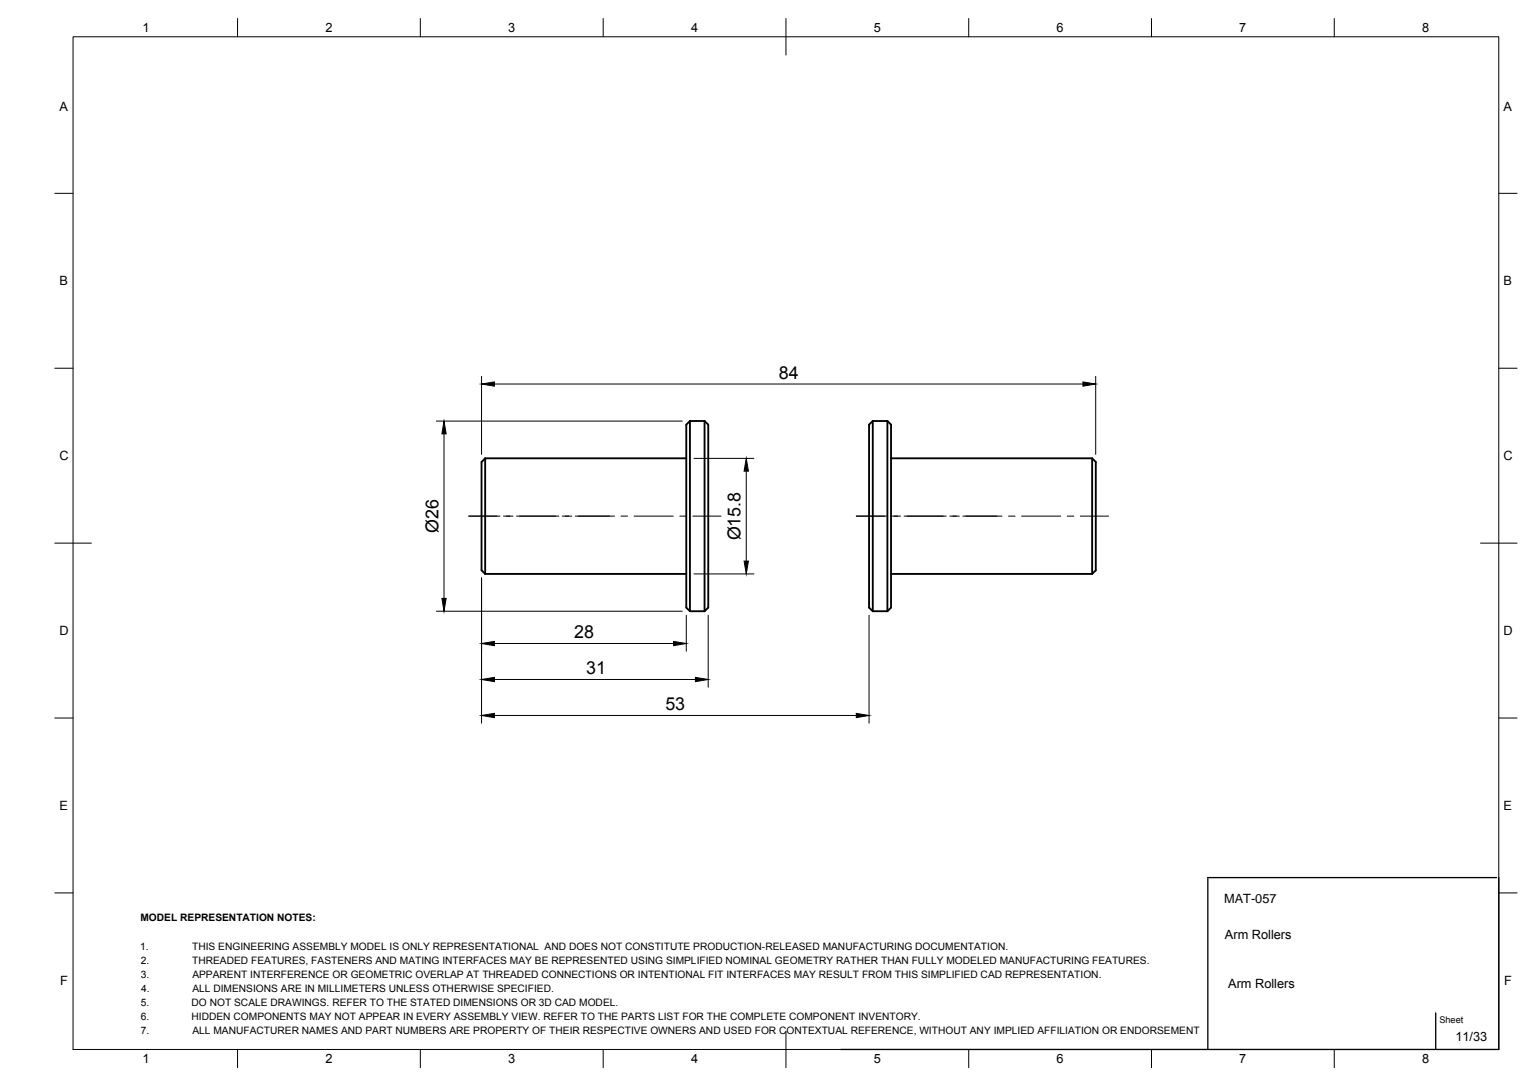
ISO-10303-21;
HEADER;
/* Generated by software containing ST-Developer
 * from STEP Tools, Inc. (www.steptools.com) 
 */

FILE_DESCRIPTION(
/* description */ ('STEP AP214', 'CAx-IF Rec.Pracs.---Representation and Presentation of Product Manufa
cturing Information (PMI)---4.0---2014-10-13'),
/* implementation_level */ '2;1');

FILE_NAME(
/* name */ 'Arm Rollers.step',
/* time_stamp */ '2026-10-28T23:34:22+01:00',
/* author */ (''),
/* organization */ (''),
/* preprocessor_version */ 'ST-DEVELOPER v20.2',
/* originating_system */ 'Autodesk Translation Framework v15.17.0.0',
/* authorisation */ '');

FILE_SCHEMA (('AP242_MANAGED_MODEL_BASED_3D_ENGINEERING_MIM_LF { 1 0 10303 442 2 1 4 }'));
ENDSEC;

DATA;
#10=MECHANICAL_DESIGN_GEOMETRIC_PRESENTATION_REPRESENTATION('',(#252,#253),#27807);
#208=SHAPE_REPRESENTATION_RELATIONSHIP('SRR','None',#27903,#230);
#230=ADVANCED_BREP_SHAPE_REPRESENTATION('',(#281,#282),#27783);
#252=STYLED_ITEM('',(#28063),#281);
#253=STYLED_ITEM('',(#28063),#282);
#281=MANIFOLD_SOLID_BREP('Body1',#12028);
#282=MANIFOLD_SOLID_BREP('Body2',#12029);
#375=FACE_BOUND('',#2200,.T.);
#376=FACE_BOUND('',#2209,.T.);
#536=PLANE('',#12763);
#537=PLANE('',#12764);
#538=PLANE('',#12765);
#539=PLANE('',#12779);
#540=PLANE('',#12780);
#541=PLANE('',#12781);
#1068=CYLINDRICAL_SURFACE('',#12760,7.89999999999999);
#1069=CYLINDRICAL_SURFACE('',#12762,13.);
#1070=CYLINDRICAL_SURFACE('',#12776,7.89999999999999);
#1071=CYLINDRICAL_SURFACE('',#12778,13.);
#1456=FACE_OUTER_BOUND('',#2193,.T.);
#1457=FACE_OUTER_BOUND('',#2194,.T.);
#1458=FACE_OUTER_BOUND('',#2195,.T.);
#1459=FACE_OUTER_BOUND('',#2196,.T.);
#1460=FACE_OUTER_BOUND('',#2197,.T.);
#1461=FACE_OUTER_BOUND('',#2198,.T.);
#1462=FACE_OUTER_BOUND('',#2199,.T.);
#1463=FACE_OUTER_BOUND('',#2201,.T.);
#1464=FACE_OUTER_BOUND('',#2202,.T.);
#1465=FACE_OUTER_BOUND('',#2203,.T.);
#1466=FACE_OUTER_BOUND('',#2204,.T.);
#1467=FACE_OUTER_BOUND('',#2205,.T.);
#1468=FACE_OUTER_BOUND('',#2206,.T.);
#1469=FACE_OUTER_BOUND('',#2207,.T.);
#1470=FACE_OUTER_BOUND('',#2208,.T.);
#1471=FACE_OUTER_BOUND('',#2210,.T.);
#2193=EDGE_LOOP('',(#8961,#8962,#8963,#8964));
#2194=EDGE_LOOP('',(#8965,#8966,#8967,#8968));
#2195=EDGE_LOOP('',(#8969,#8970,#8971,#8972,#8973));
#2196=EDGE_LOOP('',(#8974,#8975,#8976,#8977));
#2197=EDGE_LOOP('',(#8978,#8979,#8980,#8981,#8982));
#2198=EDGE_LOOP('',(#8983));
#2199=EDGE_LOOP('',(#8984));
#2200=EDGE_LOOP('',(#8985));
#2201=EDGE_LOOP('',(#8986));
#2202=EDGE_LOOP('',(#8987,#8988,#8989,#8990));
#2203=EDGE_LOOP('',(#8991,#8992,#8993,#8994));
#2204=EDGE_LOOP('',(#8995,#8996,#8997,#8998,#8999));
#2205=EDGE_LOOP('',(#9000,#9001,#9002,#9003));
#2206=EDGE_LOOP('',(#9004,#9005,#9006,#9007,#9008));
#2207=EDGE_LOOP('',(#9009));
#2208=EDGE_LOOP('',(#9010));
#2209=EDGE_LOOP('',(#9011));
#2210=EDGE_LOOP('',(#9012));
#3045=LINE('',#18795,#3865);
#3046=LINE('',#18801,#3866);
#3047=LINE('',#18809,#3867);
#3048=LINE('',#18814,#3868);
#3049=LINE('',#18816,#3869);
#3050=LINE('',#18824,#3870);
#3051=LINE('',#18830,#3871);
#3052=LINE('',#18837,#3872);
#3053=LINE('',#18843,#3873);
#3054=LINE('',#18845,#3874);
#3865=VECTOR('',#14931,7.39999999999998);
#3866=VECTOR('',#14938,12.5);
#3867=VECTOR('',#14947,13.);
#3868=VECTOR('',#14954,7.89999999999999);
#3869=VECTOR('',#14957,13.);
#3870=VECTOR('',#14968,7.39999999999998);
#3871=VECTOR('',#14975,12.5);
#3872=VECTOR('',#14982,13.);
#3873=VECTOR('',#14991,7.89999999999999);
#3874=VECTOR('',#14994,13.);
#4609=CIRCLE('',#12751,7.89999999999999);
#4610=CIRCLE('',#12752,7.39999999999998);
#4611=CIRCLE('',#12754,13.);
#4612=CIRCLE('',#12755,12.5);
#4613=CIRCLE('',#12757,13.);
#4614=CIRCLE('',#12758,13.);
#4615=CIRCLE('',#12759,12.5);
#4616=CIRCLE('',#12761,7.89999999999999);
#4617=CIRCLE('',#12767,7.89999999999999);
#4618=CIRCLE('',#12768,7.39999999999998);
#4619=CIRCLE('',#12770,13.);
#4620=CIRCLE('',#12771,12.5);
#4621=CIRCLE('',#12773,13.);
#4622=CIRCLE('',#12774,12.5);
#4623=CIRCLE('',#12775,13.);
#4624=CIRCLE('',#12777,7.89999999999999);
#5393=VERTEX_POINT('',#18792);
#5394=VERTEX_POINT('',#18794);
#5395=VERTEX_POINT('',#18798);
#5396=VERTEX_POINT('',#18800);
#5397=VERTEX_POINT('',#18804);
#5398=VERTEX_POINT('',#18805);
#5399=VERTEX_POINT('',#18808);
#5400=VERTEX_POINT('',#18812);
#5401=VERTEX_POINT('',#18821);
#5402=VERTEX_POINT('',#18823);
#5403=VERTEX_POINT('',#18827);
#5404=VERTEX_POINT('',#18829);
#5405=VERTEX_POINT('',#18833);
#5406=VERTEX_POINT('',#18834);
#5407=VERTEX_POINT('',#18836);
#5408=VERTEX_POINT('',#18841);
#6693=EDGE_CURVE('',#5393,#5393,#4609,.T.);
#6694=EDGE_CURVE('',#5393,#5394,#3045,.T.);
#6695=EDGE_CURVE('',#5394,#5394,#4610,.T.);
#6696=EDGE_CURVE('',#5395,#5395,#4611,.T.);
#6697=EDGE_CURVE('',#5395,#5396,#3046,.T.);
#6698=EDGE_CURVE('',#5396,#5396,#4612,.T.);
#6699=EDGE_CURVE('',#5397,#5398,#4613,.T.);
#6700=EDGE_CURVE('',#5398,#5397,#4614,.T.);
#6701=EDGE_CURVE('',#5398,#5399,#3047,.T.);
#6702=EDGE_CURVE('',#5399,#5399,#4615,.T.);
#6703=EDGE_CURVE('',#5400,#5400,#4616,.T.);
#6704=EDGE_CURVE('',#5400,#5393,#3048,.T.);
#6705=EDGE_CURVE('',#5397,#5395,#3049,.T.);
#6706=EDGE_CURVE('',#5401,#5401,#4617,.T.);
#6707=EDGE_CURVE('',#5401,#5402,#3050,.T.);
#6708=EDGE_CURVE('',#5402,#5402,#4618,.T.);
#6709=EDGE_CURVE('',#5403,#5403,#4619,.T.);
#6710=EDGE_CURVE('',#5403,#5404,#3051,.T.);
#6711=EDGE_CURVE('',#5404,#5404,#4620,.T.);
#6712=EDGE_CURVE('',#5405,#5406,#4621,.T.);
#6713=EDGE_CURVE('',#5406,#5407,#3052,.T.);
#6714=EDGE_CURVE('',#5407,#5407,#4622,.T.);
#6715=EDGE_CURVE('',#5406,#5405,#4623,.T.);
#6716=EDGE_CURVE('',#5408,#5408,#4624,.T.);
#6717=EDGE_CURVE('',#5408,#5401,#3053,.T.);
#6718=EDGE_CURVE('',#5405,#5403,#3054,.T.);
#8961=ORIENTED_EDGE('',*,*,#6693,.F.);
#8962=ORIENTED_EDGE('',*,*,#6694,.T.);
#8963=ORIENTED_EDGE('',*,*,#6695,.F.);
#8964=ORIENTED_EDGE('',*,*,#6694,.F.);
#8965=ORIENTED_EDGE('',*,*,#6696,.F.);
#8966=ORIENTED_EDGE('',*,*,#6697,.T.);
#8967=ORIENTED_EDGE('',*,*,#6698,.F.);
#8968=ORIENTED_EDGE('',*,*,#6697,.F.);
#8969=ORIENTED_EDGE('',*,*,#6699,.F.);
#8970=ORIENTED_EDGE('',*,*,#6700,.F.);
#8971=ORIENTED_EDGE('',*,*,#6701,.T.);
#8972=ORIENTED_EDGE('',*,*,#6702,.F.);
#8973=ORIENTED_EDGE('',*,*,#6701,.F.);
#8974=ORIENTED_EDGE('',*,*,#6703,.T.);
#8975=ORIENTED_EDGE('',*,*,#6704,.T.);
#8976=ORIENTED_EDGE('',*,*,#6693,.T.);
#8977=ORIENTED_EDGE('',*,*,#6704,.F.);
#8978=ORIENTED_EDGE('',*,*,#6699,.T.);
#8979=ORIENTED_EDGE('',*,*,#6700,.T.);
#8980=ORIENTED_EDGE('',*,*,#6705,.T.);
#8981=ORIENTED_EDGE('',*,*,#6696,.T.);
#8982=ORIENTED_EDGE('',*,*,#6705,.F.);
#8983=ORIENTED_EDGE('',*,*,#6698,.T.);
#8984=ORIENTED_EDGE('',*,*,#6702,.T.);
#8985=ORIENTED_EDGE('',*,*,#6703,.F.);
#8986=ORIENTED_EDGE('',*,*,#6695,.T.);
#8987=ORIENTED_EDGE('',*,*,#6706,.T.);
#8988=ORIENTED_EDGE('',*,*,#6707,.T.);
#8989=ORIENTED_EDGE('',*,*,#6708,.T.);
#8990=ORIENTED_EDGE('',*,*,#6707,.F.);
#8991=ORIENTED_EDGE('',*,*,#6709,.T.);
#8992=ORIENTED_EDGE('',*,*,#6710,.T.);
#8993=ORIENTED_EDGE('',*,*,#6711,.T.);
#8994=ORIENTED_EDGE('',*,*,#6710,.F.);
#8995=ORIENTED_EDGE('',*,*,#6712,.T.);
#8996=ORIENTED_EDGE('',*,*,#6713,.T.);
#8997=ORIENTED_EDGE('',*,*,#6714,.T.);
#8998=ORIENTED_EDGE('',*,*,#6713,.F.);
#8999=ORIENTED_EDGE('',*,*,#6715,.T.);
#9000=ORIENTED_EDGE('',*,*,#6716,.F.);
#9001=ORIENTED_EDGE('',*,*,#6717,.T.);
#9002=ORIENTED_EDGE('',*,*,#6706,.F.);
#9003=ORIENTED_EDGE('',*,*,#6717,.F.);
#9004=ORIENTED_EDGE('',*,*,#6712,.F.);
#9005=ORIENTED_EDGE('',*,*,#6718,.T.);
#9006=ORIENTED_EDGE('',*,*,#6709,.F.);
#9007=ORIENTED_EDGE('',*,*,#6718,.F.);
#9008=ORIENTED_EDGE('',*,*,#6715,.F.);
#9009=ORIENTED_EDGE('',*,*,#6711,.F.);
#9010=ORIENTED_EDGE('',*,*,#6714,.F.);
#9011=ORIENTED_EDGE('',*,*,#6716,.T.);
#9012=ORIENTED_EDGE('',*,*,#6708,.F.);
#11285=CONICAL_SURFACE('',#12750,7.39999999999998,0.785398163397459);
#11286=CONICAL_SURFACE('',#12753,12.5,0.785398163397438);
#11287=CONICAL_SURFACE('',#12756,13.,0.785398163397455);
#11288=CONICAL_SURFACE('',#12766,7.39999999999998,0.785398163397459);
#11289=CONICAL_SURFACE('',#12769,12.5,0.785398163397438);
#11290=CONICAL_SURFACE('',#12772,13.,0.785398163397455);
#11538=ADVANCED_FACE('',(#1456),#11285,.T.);
#11539=ADVANCED_FACE('',(#1457),#11286,.T.);
#11540=ADVANCED_FACE('',(#1458),#11287,.T.);
#11541=ADVANCED_FACE('',(#1459),#1068,.T.);
#11542=ADVANCED_FACE('',(#1460),#1069,.T.);
#11543=ADVANCED_FACE('',(#1461),#536,.T.);
#11544=ADVANCED_FACE('',(#1462,#375),#537,.F.);
#11545=ADVANCED_FACE('',(#1463),#538,.T.);
#11546=ADVANCED_FACE('',(#1464),#11288,.T.);
#11547=ADVANCED_FACE('',(#1465),#11289,.T.);
#11548=ADVANCED_FACE('',(#1466),#11290,.T.);
#11549=ADVANCED_FACE('',(#1467),#1070,.T.);
#11550=ADVANCED_FACE('',(#1468),#1071,.T.);
#11551=ADVANCED_FACE('',(#1469),#539,.T.);
#11552=ADVANCED_FACE('',(#1470,#376),#540,.F.);
#11553=ADVANCED_FACE('',(#1471),#541,.T.);
#12028=CLOSED_SHELL('',(#11538,#11539,#11540,#11541,#11542,#11543,#11544,
#11545));
#12029=CLOSED_SHELL('',(#11546,#11547,#11548,#11549,#11550,#11551,#11552,
#11553));
#12749=AXIS2_PLACEMENT_3D('',#18790,#14925,#14926);
#12750=AXIS2_PLACEMENT_3D('',#18791,#14927,#14928);
#12751=AXIS2_PLACEMENT_3D('',#18793,#14929,#14930);
#12752=AXIS2_PLACEMENT_3D('',#18796,#14932,#14933);
#12753=AXIS2_PLACEMENT_3D('',#18797,#14934,#14935);
#12754=AXIS2_PLACEMENT_3D('',#18799,#14936,#14937);
#12755=AXIS2_PLACEMENT_3D('',#18802,#14939,#14940);
#12756=AXIS2_PLACEMENT_3D('',#18803,#14941,#14942);
#12757=AXIS2_PLACEMENT_3D('',#18806,#14943,#14944);
#12758=AXIS2_PLACEMENT_3D('',#18807,#14945,#14946);
#12759=AXIS2_PLACEMENT_3D('',#18810,#14948,#14949);
#12760=AXIS2_PLACEMENT_3D('',#18811,#14950,#14951);
#12761=AXIS2_PLACEMENT_3D('',#18813,#14952,#14953);
#12762=AXIS2_PLACEMENT_3D('',#18815,#14955,#14956);
#12763=AXIS2_PLACEMENT_3D('',#18817,#14958,#14959);
#12764=AXIS2_PLACEMENT_3D('',#18818,#14960,#14961);
#12765=AXIS2_PLACEMENT_3D('',#18819,#14962,#14963);
#12766=AXIS2_PLACEMENT_3D('',#18820,#14964,#14965);
#12767=AXIS2_PLACEMENT_3D('',#18822,#14966,#14967);
#12768=AXIS2_PLACEMENT_3D('',#18825,#14969,#14970);
#12769=AXIS2_PLACEMENT_3D('',#18826,#14971,#14972);
#12770=AXIS2_PLACEMENT_3D('',#18828,#14973,#14974);
#12771=AXIS2_PLACEMENT_3D('',#18831,#14976,#14977);
#12772=AXIS2_PLACEMENT_3D('',#18832,#14978,#14979);
#12773=AXIS2_PLACEMENT_3D('',#18835,#14980,#14981);
#12774=AXIS2_PLACEMENT_3D('',#18838,#14983,#14984);
#12775=AXIS2_PLACEMENT_3D('',#18839,#14985,#14986);
#12776=AXIS2_PLACEMENT_3D('',#18840,#14987,#14988);
#12777=AXIS2_PLACEMENT_3D('',#18842,#14989,#14990);
#12778=AXIS2_PLACEMENT_3D('',#18844,#14992,#14993);
#12779=AXIS2_PLACEMENT_3D('',#18846,#14995,#14996);
#12780=AXIS2_PLACEMENT_3D('',#18847,#14997,#14998);
#12781=AXIS2_PLACEMENT_3D('',#18848,#14999,#15000);
#14925=DIRECTION('axis',(0.,0.,1.));
#14926=DIRECTION('refdir',(1.,0.,0.));
#14927=DIRECTION('center_axis',(0.,0.,1.));
#14928=DIRECTION('ref_axis',(1.,0.,0.));
#14929=DIRECTION('center_axis',(0.,0.,1.));
#14930=DIRECTION('ref_axis',(-1.,0.,0.));
#14931=DIRECTION('',(0.707106781186555,8.65956056235502E-17,-0.70710678118654));
#14932=DIRECTION('center_axis',(0.,0.,-1.));
#14933=DIRECTION('ref_axis',(-1.,0.,0.));
#14934=DIRECTION('center_axis',(0.,0.,-1.));
#14935=DIRECTION('ref_axis',(-1.,0.,0.));
#14936=DIRECTION('center_axis',(0.,0.,-1.));
#14937=DIRECTION('ref_axis',(1.,0.,0.));
#14938=DIRECTION('',(-0.70710678118654,8.65956056235484E-17,0.707106781186555));
#14939=DIRECTION('center_axis',(0.,0.,1.));
#14940=DIRECTION('ref_axis',(1.,0.,0.));
#14941=DIRECTION('center_axis',(0.,0.,1.));
#14942=DIRECTION('ref_axis',(1.,0.,0.));
#14943=DIRECTION('center_axis',(0.,0.,1.));
#14944=DIRECTION('ref_axis',(1.,0.,0.));
#14945=DIRECTION('center_axis',(0.,0.,1.));
#14946=DIRECTION('ref_axis',(1.,0.,0.));
#14947=DIRECTION('',(0.707106781186552,8.65956056235499E-17,-0.707106781186543));
#14948=DIRECTION('center_axis',(0.,0.,-1.));
#14949=DIRECTION('ref_axis',(1.,0.,0.));
#14950=DIRECTION('center_axis',(0.,0.,1.));
#14951=DIRECTION('ref_axis',(1.,0.,0.));
#14952=DIRECTION('center_axis',(0.,0.,-1.));
#14953=DIRECTION('ref_axis',(-1.,0.,0.));
#14954=DIRECTION('',(0.,0.,-1.));
#14955=DIRECTION('center_axis',(0.,0.,-1.));
#14956=DIRECTION('ref_axis',(-1.,0.,0.));
#14957=DIRECTION('',(0.,0.,1.));
#14958=DIRECTION('center_axis',(0.,0.,1.));
#14959=DIRECTION('ref_axis',(1.,0.,0.));
#14960=DIRECTION('center_axis',(0.,0.,1.));
#14961=DIRECTION('ref_axis',(1.,0.,0.));
#14962=DIRECTION('center_axis',(0.,0.,-1.));
#14963=DIRECTION('ref_axis',(1.,0.,0.));
#14964=DIRECTION('center_axis',(0.,0.,-1.));
#14965=DIRECTION('ref_axis',(1.,0.,0.));
#14966=DIRECTION('center_axis',(0.,0.,1.));
#14967=DIRECTION('ref_axis',(-1.,0.,0.));
#14968=DIRECTION('',(0.707106781186555,-8.65956056235502E-17,0.70710678118654));
#14969=DIRECTION('center_axis',(0.,0.,-1.));
#14970=DIRECTION('ref_axis',(-1.,0.,0.));
#14971=DIRECTION('center_axis',(0.,0.,1.));
#14972=DIRECTION('ref_axis',(-1.,0.,0.));
#14973=DIRECTION('center_axis',(0.,0.,-1.));
#14974=DIRECTION('ref_axis',(1.,0.,0.));
#14975=DIRECTION('',(-0.70710678118654,-8.65956056235484E-17,-0.707106781186555));
#14976=DIRECTION('center_axis',(0.,0.,1.));
#14977=DIRECTION('ref_axis',(1.,0.,0.));
#14978=DIRECTION('center_axis',(0.,0.,-1.));
#14979=DIRECTION('ref_axis',(1.,0.,0.));
#14980=DIRECTION('center_axis',(0.,0.,1.));
#14981=DIRECTION('ref_axis',(1.,0.,0.));
#14982=DIRECTION('',(0.707106781186552,-8.65956056235499E-17,0.707106781186543));
#14983=DIRECTION('center_axis',(0.,0.,-1.));
#14984=DIRECTION('ref_axis',(1.,0.,0.));
#14985=DIRECTION('center_axis',(0.,0.,1.));
#14986=DIRECTION('ref_axis',(1.,0.,0.));
#14987=DIRECTION('center_axis',(0.,0.,-1.));
#14988=DIRECTION('ref_axis',(1.,0.,0.));
#14989=DIRECTION('center_axis',(0.,0.,-1.));
#14990=DIRECTION('ref_axis',(-1.,0.,0.));
#14991=DIRECTION('',(0.,0.,1.));
#14992=DIRECTION('center_axis',(0.,0.,1.));
#14993=DIRECTION('ref_axis',(-1.,0.,0.));
#14994=DIRECTION('',(0.,0.,-1.));
#14995=DIRECTION('center_axis',(0.,0.,-1.));
#14996=DIRECTION('ref_axis',(1.,0.,0.));
#14997=DIRECTION('center_axis',(0.,0.,-1.));
#14998=DIRECTION('ref_axis',(1.,0.,0.));
#14999=DIRECTION('center_axis',(0.,0.,1.));
#15000=DIRECTION('ref_axis',(1.,0.,0.));
#18790=CARTESIAN_POINT('',(0.,0.,0.));
#18791=CARTESIAN_POINT('Origin',(37.0412526478464,187.739737607039,211.073593133701));
#18792=CARTESIAN_POINT('',(29.1412526478464,187.739737607039,211.573593133701));
#18793=CARTESIAN_POINT('Origin',(37.0412526478464,187.739737607039,211.573593133701));
#18794=CARTESIAN_POINT('',(29.6412526478464,187.739737607039,211.073593133701));
#18795=CARTESIAN_POINT('',(29.6412526478464,187.739737607039,211.073593133701));
#18796=CARTESIAN_POINT('Origin',(37.0412526478464,187.739737607039,211.073593133701));
#18797=CARTESIAN_POINT('Origin',(37.0412526479213,187.739737607024,242.073593133701));
#18798=CARTESIAN_POINT('',(50.0412526479213,187.739737607024,241.573593133701));
#18799=CARTESIAN_POINT('Origin',(37.0412526479213,187.739737607024,241.573593133701));
#18800=CARTESIAN_POINT('',(49.5412526479213,187.739737607024,242.073593133701));
#18801=CARTESIAN_POINT('',(49.5412526479213,187.739737607024,242.073593133701));
#18802=CARTESIAN_POINT('Origin',(37.0412526479213,187.739737607024,242.073593133701));
#18803=CARTESIAN_POINT('Origin',(37.0412526479213,187.739737607024,239.573593133701));
#18804=CARTESIAN_POINT('',(50.0412526479213,187.739737607024,239.573593133701));
#18805=CARTESIAN_POINT('',(24.0412526479213,187.739737607024,239.573593133701));
#18806=CARTESIAN_POINT('Origin',(37.0412526479213,187.739737607024,239.573593133701));
#18807=CARTESIAN_POINT('Origin',(37.0412526479213,187.739737607024,239.573593133701));
#18808=CARTESIAN_POINT('',(24.5412526479213,187.739737607024,239.073593133701));
#18809=CARTESIAN_POINT('',(24.0412526479213,187.739737607024,239.573593133701));
#18810=CARTESIAN_POINT('Origin',(37.0412526479213,187.739737607024,239.073593133701));
#18811=CARTESIAN_POINT('Origin',(37.0412526478464,187.739737607039,188.729018848206));
#18812=CARTESIAN_POINT('',(29.1412526478464,187.739737607039,239.073593133701));
#18813=CARTESIAN_POINT('Origin',(37.0412526478464,187.739737607039,239.073593133701));
#18814=CARTESIAN_POINT('',(29.1412526478464,187.739737607039,188.729018848206));
#18815=CARTESIAN_POINT('Origin',(37.0412526479213,187.739737607024,242.073593133701));
#18816=CARTESIAN_POINT('',(50.0412526479213,187.739737607024,242.073593133701));
#18817=CARTESIAN_POINT('Origin',(37.0412526479213,187.739737607024,242.073593133701));
#18818=CARTESIAN_POINT('Origin',(37.0412526479213,187.739737607024,239.073593133701));
#18819=CARTESIAN_POINT('Origin',(-276.958747352154,52.7397376070391,211.073593133701));
#18820=CARTESIAN_POINT('Origin',(37.0412526478464,187.739737607039,295.073593133701));
#18821=CARTESIAN_POINT('',(29.1412526478464,187.739737607039,294.573593133701));
#18822=CARTESIAN_POINT('Origin',(37.0412526478464,187.739737607039,294.573593133701));
#18823=CARTESIAN_POINT('',(29.6412526478464,187.739737607039,295.073593133701));
#18824=CARTESIAN_POINT('',(29.6412526478464,187.739737607039,295.073593133701));
#18825=CARTESIAN_POINT('Origin',(37.0412526478464,187.739737607039,295.073593133701));
#18826=CARTESIAN_POINT('Origin',(37.0412526479213,187.739737607024,264.073593133701));
#18827=CARTESIAN_POINT('',(50.0412526479213,187.739737607024,264.573593133701));
#18828=CARTESIAN_POINT('Origin',(37.0412526479213,187.739737607024,264.573593133701));
#18829=CARTESIAN_POINT('',(49.5412526479213,187.739737607024,264.073593133701));
#18830=CARTESIAN_POINT('',(49.5412526479213,187.739737607024,264.073593133701));
#18831=CARTESIAN_POINT('Origin',(37.0412526479213,187.739737607024,264.073593133701));
#18832=CARTESIAN_POINT('Origin',(37.0412526479213,187.739737607024,266.573593133701));
#18833=CARTESIAN_POINT('',(50.0412526479213,187.739737607024,266.573593133701));
#18834=CARTESIAN_POINT('',(24.0412526479213,187.739737607024,266.573593133701));
#18835=CARTESIAN_POINT('Origin',(37.0412526479213,187.739737607024,266.573593133701));
#18836=CARTESIAN_POINT('',(24.5412526479213,187.739737607024,267.073593133701));
#18837=CARTESIAN_POINT('',(24.0412526479213,187.739737607024,266.573593133701));
#18838=CARTESIAN_POINT('Origin',(37.0412526479213,187.739737607024,267.073593133701));
#18839=CARTESIAN_POINT('Origin',(37.0412526479213,187.739737607024,266.573593133701));
#18840=CARTESIAN_POINT('Origin',(37.0412526478464,187.739737607039,317.418167419196));
#18841=CARTESIAN_POINT('',(29.1412526478464,187.739737607039,267.073593133701));
#18842=CARTESIAN_POINT('Origin',(37.0412526478464,187.739737607039,267.073593133701));
#18843=CARTESIAN_POINT('',(29.1412526478464,187.739737607039,317.418167419196));
#18844=CARTESIAN_POINT('Origin',(37.0412526479213,187.739737607024,264.073593133701));
#18845=CARTESIAN_POINT('',(50.0412526479213,187.739737607024,264.073593133701));
#18846=CARTESIAN_POINT('Origin',(37.0412526479213,187.739737607024,264.073593133701));
#18847=CARTESIAN_POINT('Origin',(37.0412526479213,187.739737607024,267.073593133701));
#18848=CARTESIAN_POINT('Origin',(-276.958747352154,52.7397376070391,295.073593133701));
#27754=UNCERTAINTY_MEASURE_WITH_UNIT(LENGTH_MEASURE(0.01),#27808,
'DISTANCE_ACCURACY_VALUE',
'Maximum model space distance between geometric entities at asserted c
onnectivities');
#27778=UNCERTAINTY_MEASURE_WITH_UNIT(LENGTH_MEASURE(0.01),#27808,
'DISTANCE_ACCURACY_VALUE',
'Maximum model space distance between geometric entities at asserted c
onnectivities');
#27783=(
GEOMETRIC_REPRESENTATION_CONTEXT(3)
GLOBAL_UNCERTAINTY_ASSIGNED_CONTEXT((#27754))
GLOBAL_UNIT_ASSIGNED_CONTEXT((#27808,#27810,#27811))
REPRESENTATION_CONTEXT('','3D')
);
#27807=(
GEOMETRIC_REPRESENTATION_CONTEXT(3)
GLOBAL_UNCERTAINTY_ASSIGNED_CONTEXT((#27778))
GLOBAL_UNIT_ASSIGNED_CONTEXT((#27808,#27810,#27811))
REPRESENTATION_CONTEXT('','3D')
);
#27808=(
LENGTH_UNIT()
NAMED_UNIT(*)
SI_UNIT(.MILLI.,.METRE.)
);
#27810=(
NAMED_UNIT(*)
PLANE_ANGLE_UNIT()
SI_UNIT($,.RADIAN.)
);
#27811=(
NAMED_UNIT(*)
SI_UNIT($,.STERADIAN.)
SOLID_ANGLE_UNIT()
);
#27816=SHAPE_DEFINITION_REPRESENTATION(#27844,#27903);
#27844=PRODUCT_DEFINITION_SHAPE('',$,#27932);
#27903=SHAPE_REPRESENTATION('',(#12749),#27783);
#27927=PRODUCT_DEFINITION_CONTEXT('part definition',#28013,'design');
#27932=PRODUCT_DEFINITION('Arm Rollers','Arm Rollers',#27960,#27927);
#27960=PRODUCT_DEFINITION_FORMATION('',$,#28019);
#28013=APPLICATION_CONTEXT('Managed model based 3d engineering');
#28014=PRODUCT_CONTEXT('part definition',#28013,'mechanical');
#28019=PRODUCT('Arm Rollers','Arm Rollers',$,(#28014));
#28057=COLOUR_RGB('Light Blue',0.38,0.62,0.78);
#28058=FILL_AREA_STYLE_COLOUR('',#28057);
#28059=FILL_AREA_STYLE('',(#28058));
#28060=SURFACE_STYLE_FILL_AREA(#28059);
#28061=SURFACE_SIDE_STYLE('',(#28060));
#28062=SURFACE_STYLE_USAGE(.BOTH.,#28061);
#28063=PRESENTATION_STYLE_ASSIGNMENT((#28062));
ENDSEC;
END-ISO-10303-21;
